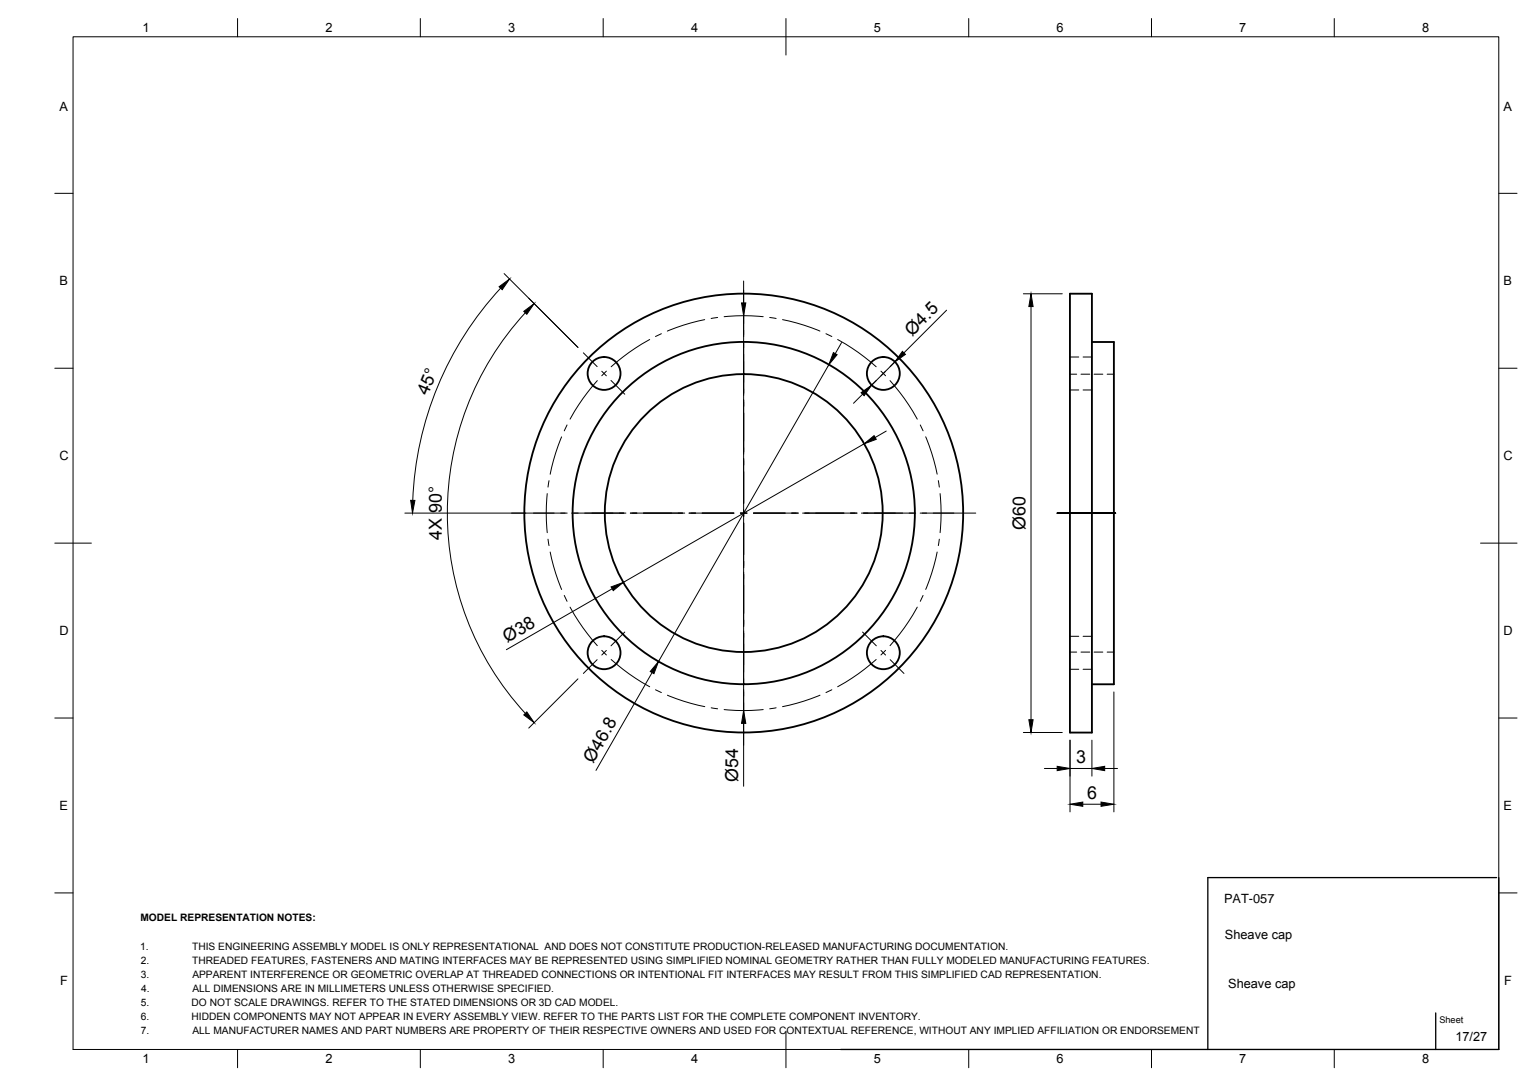
ISO-10303-21;
HEADER;
/* Generated by software containing ST-Developer
 * from STEP Tools, Inc. (www.steptools.com) 
 */

FILE_DESCRIPTION(
/* description */ ('Bearing-mounted hook block'),
/* implementation_level */ '2;1');

FILE_NAME(
/* name */ 'Sheave cap.step',
/* time_stamp */ '2026-10-28T22:30:11-07:00',
/* author */ (''),
/* organization */ (''),
/* preprocessor_version */ 'ST-DEVELOPER v20.2',
/* originating_system */ 'Autodesk Translation Framework v15.17.0.0',
/* authorisation */ '');

FILE_SCHEMA (('AUTOMOTIVE_DESIGN { 1 0 10303 214 3 1 1 }'));
ENDSEC;

DATA;
#10=MECHANICAL_DESIGN_GEOMETRIC_PRESENTATION_REPRESENTATION('',(#350),#7609);
#294=SHAPE_REPRESENTATION_RELATIONSHIP('SRR','None',#7743,#318);
#318=ADVANCED_BREP_SHAPE_REPRESENTATION('',(#380),#7603);
#350=STYLED_ITEM('',(#7945),#380);
#380=MANIFOLD_SOLID_BREP('Body1',#3948);
#541=LINE('',#7289,#771);
#542=LINE('',#7295,#772);
#543=LINE('',#7301,#773);
#544=LINE('',#7307,#774);
#545=LINE('',#7313,#775);
#546=LINE('',#7320,#776);
#547=LINE('',#7326,#777);
#771=VECTOR('',#5756,0.225);
#772=VECTOR('',#5763,0.225);
#773=VECTOR('',#5770,0.225);
#774=VECTOR('',#5777,0.225);
#775=VECTOR('',#5784,2.34);
#776=VECTOR('',#5793,1.9);
#777=VECTOR('',#5800,3.);
#904=CYLINDRICAL_SURFACE('',#4638,0.225);
#905=CYLINDRICAL_SURFACE('',#4641,0.225);
#906=CYLINDRICAL_SURFACE('',#4644,0.225);
#907=CYLINDRICAL_SURFACE('',#4647,0.225);
#908=CYLINDRICAL_SURFACE('',#4650,2.34);
#909=CYLINDRICAL_SURFACE('',#4655,1.9);
#910=CYLINDRICAL_SURFACE('',#4657,3.);
#983=FACE_BOUND('',#1486,.T.);
#984=FACE_BOUND('',#1490,.T.);
#985=FACE_BOUND('',#1491,.T.);
#986=FACE_BOUND('',#1492,.T.);
#987=FACE_BOUND('',#1493,.T.);
#988=FACE_BOUND('',#1494,.T.);
#989=FACE_BOUND('',#1496,.T.);
#990=FACE_BOUND('',#1497,.T.);
#991=FACE_BOUND('',#1498,.T.);
#992=FACE_BOUND('',#1499,.T.);
#993=FACE_BOUND('',#1500,.T.);
#1182=FACE_OUTER_BOUND('',#1480,.T.);
#1183=FACE_OUTER_BOUND('',#1481,.T.);
#1184=FACE_OUTER_BOUND('',#1482,.T.);
#1185=FACE_OUTER_BOUND('',#1483,.T.);
#1186=FACE_OUTER_BOUND('',#1484,.T.);
#1187=FACE_OUTER_BOUND('',#1485,.T.);
#1188=FACE_OUTER_BOUND('',#1487,.T.);
#1189=FACE_OUTER_BOUND('',#1488,.T.);
#1190=FACE_OUTER_BOUND('',#1489,.T.);
#1191=FACE_OUTER_BOUND('',#1495,.T.);
#1480=EDGE_LOOP('',(#3336,#3337,#3338,#3339));
#1481=EDGE_LOOP('',(#3340,#3341,#3342,#3343));
#1482=EDGE_LOOP('',(#3344,#3345,#3346,#3347));
#1483=EDGE_LOOP('',(#3348,#3349,#3350,#3351));
#1484=EDGE_LOOP('',(#3352,#3353,#3354,#3355));
#1485=EDGE_LOOP('',(#3356));
#1486=EDGE_LOOP('',(#3357));
#1487=EDGE_LOOP('',(#3358,#3359,#3360,#3361));
#1488=EDGE_LOOP('',(#3362,#3363,#3364,#3365));
#1489=EDGE_LOOP('',(#3366));
#1490=EDGE_LOOP('',(#3367));
#1491=EDGE_LOOP('',(#3368));
#1492=EDGE_LOOP('',(#3369));
#1493=EDGE_LOOP('',(#3370));
#1494=EDGE_LOOP('',(#3371));
#1495=EDGE_LOOP('',(#3372));
#1496=EDGE_LOOP('',(#3373));
#1497=EDGE_LOOP('',(#3374));
#1498=EDGE_LOOP('',(#3375));
#1499=EDGE_LOOP('',(#3376));
#1500=EDGE_LOOP('',(#3377));
#1739=CIRCLE('',#4639,0.225);
#1740=CIRCLE('',#4640,0.225);
#1741=CIRCLE('',#4642,0.225);
#1742=CIRCLE('',#4643,0.225);
#1743=CIRCLE('',#4645,0.225);
#1744=CIRCLE('',#4646,0.225);
#1745=CIRCLE('',#4648,0.225);
#1746=CIRCLE('',#4649,0.225);
#1747=CIRCLE('',#4651,2.34);
#1748=CIRCLE('',#4652,2.34);
#1749=CIRCLE('',#4654,1.9);
#1750=CIRCLE('',#4656,1.9);
#1751=CIRCLE('',#4658,3.);
#1752=CIRCLE('',#4659,3.);
#2032=VERTEX_POINT('',#7286);
#2033=VERTEX_POINT('',#7288);
#2034=VERTEX_POINT('',#7292);
#2035=VERTEX_POINT('',#7294);
#2036=VERTEX_POINT('',#7298);
#2037=VERTEX_POINT('',#7300);
#2038=VERTEX_POINT('',#7304);
#2039=VERTEX_POINT('',#7306);
#2040=VERTEX_POINT('',#7310);
#2041=VERTEX_POINT('',#7312);
#2042=VERTEX_POINT('',#7316);
#2043=VERTEX_POINT('',#7319);
#2044=VERTEX_POINT('',#7323);
#2045=VERTEX_POINT('',#7325);
#2478=EDGE_CURVE('',#2032,#2032,#1739,.T.);
#2479=EDGE_CURVE('',#2032,#2033,#541,.T.);
#2480=EDGE_CURVE('',#2033,#2033,#1740,.T.);
#2481=EDGE_CURVE('',#2034,#2034,#1741,.T.);
#2482=EDGE_CURVE('',#2034,#2035,#542,.T.);
#2483=EDGE_CURVE('',#2035,#2035,#1742,.T.);
#2484=EDGE_CURVE('',#2036,#2036,#1743,.T.);
#2485=EDGE_CURVE('',#2036,#2037,#543,.T.);
#2486=EDGE_CURVE('',#2037,#2037,#1744,.T.);
#2487=EDGE_CURVE('',#2038,#2038,#1745,.T.);
#2488=EDGE_CURVE('',#2038,#2039,#544,.T.);
#2489=EDGE_CURVE('',#2039,#2039,#1746,.T.);
#2490=EDGE_CURVE('',#2040,#2040,#1747,.T.);
#2491=EDGE_CURVE('',#2040,#2041,#545,.T.);
#2492=EDGE_CURVE('',#2041,#2041,#1748,.T.);
#2493=EDGE_CURVE('',#2042,#2042,#1749,.T.);
#2494=EDGE_CURVE('',#2042,#2043,#546,.T.);
#2495=EDGE_CURVE('',#2043,#2043,#1750,.T.);
#2496=EDGE_CURVE('',#2044,#2044,#1751,.T.);
#2497=EDGE_CURVE('',#2044,#2045,#547,.T.);
#2498=EDGE_CURVE('',#2045,#2045,#1752,.T.);
#3336=ORIENTED_EDGE('',*,*,#2478,.F.);
#3337=ORIENTED_EDGE('',*,*,#2479,.T.);
#3338=ORIENTED_EDGE('',*,*,#2480,.F.);
#3339=ORIENTED_EDGE('',*,*,#2479,.F.);
#3340=ORIENTED_EDGE('',*,*,#2481,.F.);
#3341=ORIENTED_EDGE('',*,*,#2482,.T.);
#3342=ORIENTED_EDGE('',*,*,#2483,.F.);
#3343=ORIENTED_EDGE('',*,*,#2482,.F.);
#3344=ORIENTED_EDGE('',*,*,#2484,.F.);
#3345=ORIENTED_EDGE('',*,*,#2485,.T.);
#3346=ORIENTED_EDGE('',*,*,#2486,.F.);
#3347=ORIENTED_EDGE('',*,*,#2485,.F.);
#3348=ORIENTED_EDGE('',*,*,#2487,.F.);
#3349=ORIENTED_EDGE('',*,*,#2488,.T.);
#3350=ORIENTED_EDGE('',*,*,#2489,.F.);
#3351=ORIENTED_EDGE('',*,*,#2488,.F.);
#3352=ORIENTED_EDGE('',*,*,#2490,.F.);
#3353=ORIENTED_EDGE('',*,*,#2491,.T.);
#3354=ORIENTED_EDGE('',*,*,#2492,.F.);
#3355=ORIENTED_EDGE('',*,*,#2491,.F.);
#3356=ORIENTED_EDGE('',*,*,#2490,.T.);
#3357=ORIENTED_EDGE('',*,*,#2493,.T.);
#3358=ORIENTED_EDGE('',*,*,#2493,.F.);
#3359=ORIENTED_EDGE('',*,*,#2494,.T.);
#3360=ORIENTED_EDGE('',*,*,#2495,.T.);
#3361=ORIENTED_EDGE('',*,*,#2494,.F.);
#3362=ORIENTED_EDGE('',*,*,#2496,.F.);
#3363=ORIENTED_EDGE('',*,*,#2497,.T.);
#3364=ORIENTED_EDGE('',*,*,#2498,.T.);
#3365=ORIENTED_EDGE('',*,*,#2497,.F.);
#3366=ORIENTED_EDGE('',*,*,#2496,.T.);
#3367=ORIENTED_EDGE('',*,*,#2492,.T.);
#3368=ORIENTED_EDGE('',*,*,#2489,.T.);
#3369=ORIENTED_EDGE('',*,*,#2486,.T.);
#3370=ORIENTED_EDGE('',*,*,#2483,.T.);
#3371=ORIENTED_EDGE('',*,*,#2480,.T.);
#3372=ORIENTED_EDGE('',*,*,#2498,.F.);
#3373=ORIENTED_EDGE('',*,*,#2495,.F.);
#3374=ORIENTED_EDGE('',*,*,#2487,.T.);
#3375=ORIENTED_EDGE('',*,*,#2484,.T.);
#3376=ORIENTED_EDGE('',*,*,#2481,.T.);
#3377=ORIENTED_EDGE('',*,*,#2478,.T.);
#3648=PLANE('',#4653);
#3649=PLANE('',#4660);
#3650=PLANE('',#4661);
#3864=ADVANCED_FACE('',(#1182),#904,.F.);
#3865=ADVANCED_FACE('',(#1183),#905,.F.);
#3866=ADVANCED_FACE('',(#1184),#906,.F.);
#3867=ADVANCED_FACE('',(#1185),#907,.F.);
#3868=ADVANCED_FACE('',(#1186),#908,.T.);
#3869=ADVANCED_FACE('',(#1187,#983),#3648,.T.);
#3870=ADVANCED_FACE('',(#1188),#909,.F.);
#3871=ADVANCED_FACE('',(#1189),#910,.T.);
#3872=ADVANCED_FACE('',(#1190,#984,#985,#986,#987,#988),#3649,.T.);
#3873=ADVANCED_FACE('',(#1191,#989,#990,#991,#992,#993),#3650,.F.);
#3948=CLOSED_SHELL('',(#3864,#3865,#3866,#3867,#3868,#3869,#3870,#3871,
#3872,#3873));
#4637=AXIS2_PLACEMENT_3D('',#7284,#5750,#5751);
#4638=AXIS2_PLACEMENT_3D('',#7285,#5752,#5753);
#4639=AXIS2_PLACEMENT_3D('',#7287,#5754,#5755);
#4640=AXIS2_PLACEMENT_3D('',#7290,#5757,#5758);
#4641=AXIS2_PLACEMENT_3D('',#7291,#5759,#5760);
#4642=AXIS2_PLACEMENT_3D('',#7293,#5761,#5762);
#4643=AXIS2_PLACEMENT_3D('',#7296,#5764,#5765);
#4644=AXIS2_PLACEMENT_3D('',#7297,#5766,#5767);
#4645=AXIS2_PLACEMENT_3D('',#7299,#5768,#5769);
#4646=AXIS2_PLACEMENT_3D('',#7302,#5771,#5772);
#4647=AXIS2_PLACEMENT_3D('',#7303,#5773,#5774);
#4648=AXIS2_PLACEMENT_3D('',#7305,#5775,#5776);
#4649=AXIS2_PLACEMENT_3D('',#7308,#5778,#5779);
#4650=AXIS2_PLACEMENT_3D('',#7309,#5780,#5781);
#4651=AXIS2_PLACEMENT_3D('',#7311,#5782,#5783);
#4652=AXIS2_PLACEMENT_3D('',#7314,#5785,#5786);
#4653=AXIS2_PLACEMENT_3D('',#7315,#5787,#5788);
#4654=AXIS2_PLACEMENT_3D('',#7317,#5789,#5790);
#4655=AXIS2_PLACEMENT_3D('',#7318,#5791,#5792);
#4656=AXIS2_PLACEMENT_3D('',#7321,#5794,#5795);
#4657=AXIS2_PLACEMENT_3D('',#7322,#5796,#5797);
#4658=AXIS2_PLACEMENT_3D('',#7324,#5798,#5799);
#4659=AXIS2_PLACEMENT_3D('',#7327,#5801,#5802);
#4660=AXIS2_PLACEMENT_3D('',#7328,#5803,#5804);
#4661=AXIS2_PLACEMENT_3D('',#7329,#5805,#5806);
#5750=DIRECTION('axis',(0.,0.,1.));
#5751=DIRECTION('refdir',(1.,0.,0.));
#5752=DIRECTION('center_axis',(0.,1.,0.));
#5753=DIRECTION('ref_axis',(1.,0.,0.));
#5754=DIRECTION('center_axis',(0.,1.,0.));
#5755=DIRECTION('ref_axis',(1.,0.,0.));
#5756=DIRECTION('',(0.,1.,0.));
#5757=DIRECTION('center_axis',(0.,-1.,0.));
#5758=DIRECTION('ref_axis',(1.,0.,0.));
#5759=DIRECTION('center_axis',(0.,1.,0.));
#5760=DIRECTION('ref_axis',(1.,0.,0.));
#5761=DIRECTION('center_axis',(0.,1.,0.));
#5762=DIRECTION('ref_axis',(1.,0.,0.));
#5763=DIRECTION('',(0.,1.,0.));
#5764=DIRECTION('center_axis',(0.,-1.,0.));
#5765=DIRECTION('ref_axis',(1.,0.,0.));
#5766=DIRECTION('center_axis',(0.,1.,0.));
#5767=DIRECTION('ref_axis',(1.,0.,0.));
#5768=DIRECTION('center_axis',(0.,1.,0.));
#5769=DIRECTION('ref_axis',(1.,0.,0.));
#5770=DIRECTION('',(0.,1.,0.));
#5771=DIRECTION('center_axis',(0.,-1.,0.));
#5772=DIRECTION('ref_axis',(1.,0.,0.));
#5773=DIRECTION('center_axis',(0.,1.,0.));
#5774=DIRECTION('ref_axis',(1.,0.,0.));
#5775=DIRECTION('center_axis',(0.,1.,0.));
#5776=DIRECTION('ref_axis',(1.,0.,0.));
#5777=DIRECTION('',(0.,1.,0.));
#5778=DIRECTION('center_axis',(0.,-1.,0.));
#5779=DIRECTION('ref_axis',(1.,0.,0.));
#5780=DIRECTION('center_axis',(0.,1.,0.));
#5781=DIRECTION('ref_axis',(1.,0.,0.));
#5782=DIRECTION('center_axis',(0.,1.,0.));
#5783=DIRECTION('ref_axis',(1.,0.,0.));
#5784=DIRECTION('',(0.,-1.,0.));
#5785=DIRECTION('center_axis',(0.,-1.,0.));
#5786=DIRECTION('ref_axis',(1.,0.,0.));
#5787=DIRECTION('center_axis',(0.,1.,0.));
#5788=DIRECTION('ref_axis',(1.,0.,0.));
#5789=DIRECTION('center_axis',(0.,-1.,0.));
#5790=DIRECTION('ref_axis',(1.,0.,0.));
#5791=DIRECTION('center_axis',(0.,1.,0.));
#5792=DIRECTION('ref_axis',(1.,0.,0.));
#5793=DIRECTION('',(0.,-1.,0.));
#5794=DIRECTION('center_axis',(0.,-1.,0.));
#5795=DIRECTION('ref_axis',(1.,0.,0.));
#5796=DIRECTION('center_axis',(0.,1.,0.));
#5797=DIRECTION('ref_axis',(1.,0.,0.));
#5798=DIRECTION('center_axis',(0.,1.,0.));
#5799=DIRECTION('ref_axis',(1.,0.,0.));
#5800=DIRECTION('',(0.,-1.,0.));
#5801=DIRECTION('center_axis',(0.,1.,0.));
#5802=DIRECTION('ref_axis',(1.,0.,0.));
#5803=DIRECTION('center_axis',(0.,1.,0.));
#5804=DIRECTION('ref_axis',(1.,0.,0.));
#5805=DIRECTION('center_axis',(0.,1.,0.));
#5806=DIRECTION('ref_axis',(1.,0.,0.));
#7284=CARTESIAN_POINT('',(0.,0.,0.));
#7285=CARTESIAN_POINT('Origin',(-1.90918830920368,-2.4,10.0908116907963));
#7286=CARTESIAN_POINT('',(-2.13418830920368,-2.3,10.0908116907963));
#7287=CARTESIAN_POINT('Origin',(-1.90918830920368,-2.3,10.0908116907963));
#7288=CARTESIAN_POINT('',(-2.13418830920368,-2.,10.0908116907963));
#7289=CARTESIAN_POINT('',(-2.13418830920368,-2.4,10.0908116907963));
#7290=CARTESIAN_POINT('Origin',(-1.90918830920368,-2.,10.0908116907963));
#7291=CARTESIAN_POINT('Origin',(-1.90918830920368,-2.4,13.9091883092037));
#7292=CARTESIAN_POINT('',(-2.13418830920368,-2.3,13.9091883092037));
#7293=CARTESIAN_POINT('Origin',(-1.90918830920368,-2.3,13.9091883092037));
#7294=CARTESIAN_POINT('',(-2.13418830920368,-2.,13.9091883092037));
#7295=CARTESIAN_POINT('',(-2.13418830920368,-2.4,13.9091883092037));
#7296=CARTESIAN_POINT('Origin',(-1.90918830920368,-2.,13.9091883092037));
#7297=CARTESIAN_POINT('Origin',(1.90918830920368,-2.4,13.9091883092037));
#7298=CARTESIAN_POINT('',(1.68418830920368,-2.3,13.9091883092037));
#7299=CARTESIAN_POINT('Origin',(1.90918830920368,-2.3,13.9091883092037));
#7300=CARTESIAN_POINT('',(1.68418830920368,-2.,13.9091883092037));
#7301=CARTESIAN_POINT('',(1.68418830920368,-2.4,13.9091883092037));
#7302=CARTESIAN_POINT('Origin',(1.90918830920368,-2.,13.9091883092037));
#7303=CARTESIAN_POINT('Origin',(1.90918830920368,-2.4,10.0908116907963));
#7304=CARTESIAN_POINT('',(1.68418830920368,-2.3,10.0908116907963));
#7305=CARTESIAN_POINT('Origin',(1.90918830920368,-2.3,10.0908116907963));
#7306=CARTESIAN_POINT('',(1.68418830920368,-2.,10.0908116907963));
#7307=CARTESIAN_POINT('',(1.68418830920368,-2.4,10.0908116907963));
#7308=CARTESIAN_POINT('Origin',(1.90918830920368,-2.,10.0908116907963));
#7309=CARTESIAN_POINT('Origin',(0.,-2.,12.));
#7310=CARTESIAN_POINT('',(-2.34,-1.7,12.));
#7311=CARTESIAN_POINT('Origin',(0.,-1.7,12.));
#7312=CARTESIAN_POINT('',(-2.34,-2.,12.));
#7313=CARTESIAN_POINT('',(-2.34,-2.,12.));
#7314=CARTESIAN_POINT('Origin',(0.,-2.,12.));
#7315=CARTESIAN_POINT('Origin',(0.,-1.7,12.));
#7316=CARTESIAN_POINT('',(-1.9,-1.7,12.));
#7317=CARTESIAN_POINT('Origin',(0.,-1.7,12.));
#7318=CARTESIAN_POINT('Origin',(0.,-2.3,12.));
#7319=CARTESIAN_POINT('',(-1.9,-2.3,12.));
#7320=CARTESIAN_POINT('',(-1.9,-2.3,12.));
#7321=CARTESIAN_POINT('Origin',(0.,-2.3,12.));
#7322=CARTESIAN_POINT('Origin',(0.,-2.3,12.));
#7323=CARTESIAN_POINT('',(-3.,-2.,12.));
#7324=CARTESIAN_POINT('Origin',(0.,-2.,12.));
#7325=CARTESIAN_POINT('',(-3.,-2.3,12.));
#7326=CARTESIAN_POINT('',(-3.,-2.3,12.));
#7327=CARTESIAN_POINT('Origin',(0.,-2.3,12.));
#7328=CARTESIAN_POINT('Origin',(0.,-2.,12.));
#7329=CARTESIAN_POINT('Origin',(0.,-2.3,12.));
#7573=UNCERTAINTY_MEASURE_WITH_UNIT(LENGTH_MEASURE(0.001),#7610,
'DISTANCE_ACCURACY_VALUE',
'Maximum model space distance between geometric entities at asserted c
onnectivities');
#7579=UNCERTAINTY_MEASURE_WITH_UNIT(LENGTH_MEASURE(0.001),#7610,
'DISTANCE_ACCURACY_VALUE',
'Maximum model space distance between geometric entities at asserted c
onnectivities');
#7603=(
GEOMETRIC_REPRESENTATION_CONTEXT(3)
GLOBAL_UNCERTAINTY_ASSIGNED_CONTEXT((#7573))
GLOBAL_UNIT_ASSIGNED_CONTEXT((#7610,#7612,#7613))
REPRESENTATION_CONTEXT('','3D')
);
#7609=(
GEOMETRIC_REPRESENTATION_CONTEXT(3)
GLOBAL_UNCERTAINTY_ASSIGNED_CONTEXT((#7579))
GLOBAL_UNIT_ASSIGNED_CONTEXT((#7610,#7612,#7613))
REPRESENTATION_CONTEXT('','3D')
);
#7610=(
LENGTH_UNIT()
NAMED_UNIT(*)
SI_UNIT(.CENTI.,.METRE.)
);
#7612=(
NAMED_UNIT(*)
PLANE_ANGLE_UNIT()
SI_UNIT($,.RADIAN.)
);
#7613=(
NAMED_UNIT(*)
SI_UNIT($,.STERADIAN.)
SOLID_ANGLE_UNIT()
);
#7637=SHAPE_DEFINITION_REPRESENTATION(#7694,#7743);
#7694=PRODUCT_DEFINITION_SHAPE('',$,#7773);
#7743=SHAPE_REPRESENTATION('',(#4637),#7603);
#7749=PRODUCT_DEFINITION_CONTEXT('part definition',#7838,'design');
#7773=PRODUCT_DEFINITION('Sheave cap','Sheave cap',#7802,#7749);
#7802=PRODUCT_DEFINITION_FORMATION('',$,#7863);
#7838=APPLICATION_CONTEXT(
'Core Data for Automotive Mechanical Design Process');
#7839=PRODUCT_CONTEXT('part definition',#7838,'mechanical');
#7863=PRODUCT('Sheave cap','Sheave cap','Sheave cap',(#7839));
#7939=COLOUR_RGB('Off White',0.89,0.88,0.83);
#7940=FILL_AREA_STYLE_COLOUR('',#7939);
#7941=FILL_AREA_STYLE('',(#7940));
#7942=SURFACE_STYLE_FILL_AREA(#7941);
#7943=SURFACE_SIDE_STYLE('',(#7942));
#7944=SURFACE_STYLE_USAGE(.BOTH.,#7943);
#7945=PRESENTATION_STYLE_ASSIGNMENT((#7944));
ENDSEC;
END-ISO-10303-21;
